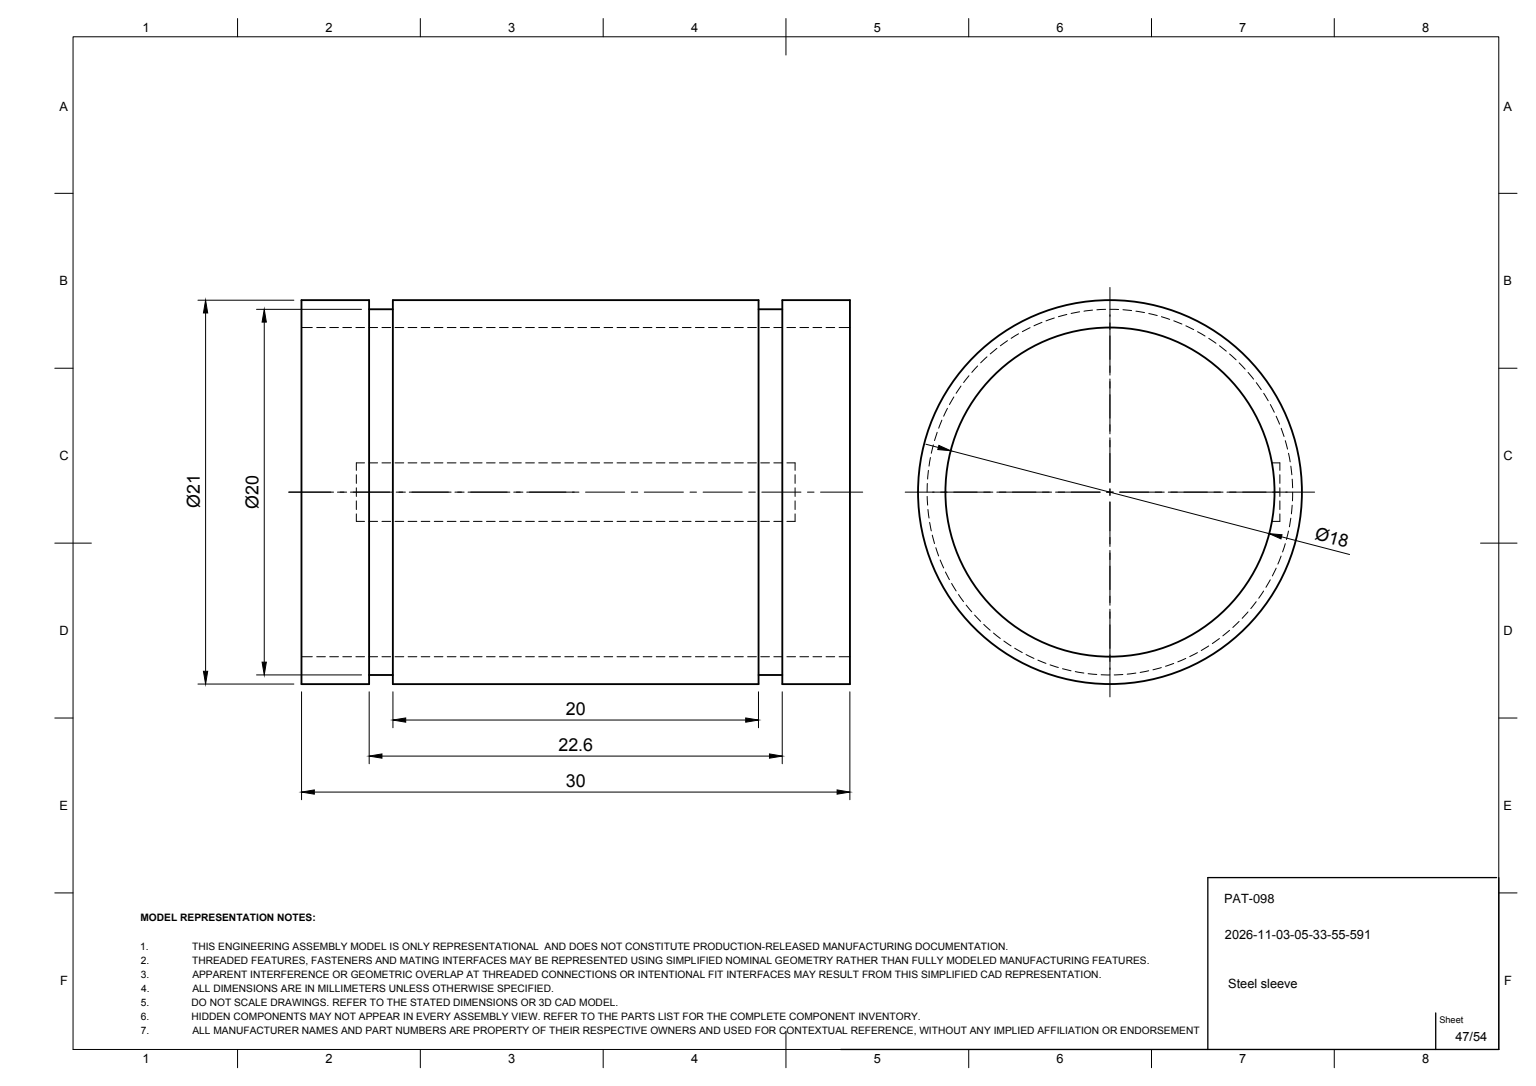
ISO-10303-21;
HEADER;
/* Generated by software containing ST-Developer
 * from STEP Tools, Inc. (www.steptools.com) 
 */

FILE_DESCRIPTION(
/* description */ ('Spring compression tester'),
/* implementation_level */ '2;1');

FILE_NAME(
/* name */ 'Steel sleeve.step',
/* time_stamp */ '2026-10-28T03:24:11-07:00',
/* author */ (''),
/* organization */ (''),
/* preprocessor_version */ 'ST-DEVELOPER v20.2',
/* originating_system */ 'Autodesk Translation Framework v15.17.0.0',
/* authorisation */ '');

FILE_SCHEMA (('AUTOMOTIVE_DESIGN { 1 0 10303 214 3 1 1 }'));
ENDSEC;

DATA;
#10=MECHANICAL_DESIGN_GEOMETRIC_PRESENTATION_REPRESENTATION('',(#1164),#43521);
#1029=SHAPE_REPRESENTATION_RELATIONSHIP('SRR','None',#43845,#1089);
#1089=ADVANCED_BREP_SHAPE_REPRESENTATION('',(#1235),#43505);
#1164=STYLED_ITEM('',(#44216),#1235);
#1235=MANIFOLD_SOLID_BREP('Body1',#18605);
#1542=FACE_BOUND('',#4256,.T.);
#1543=FACE_BOUND('',#4259,.T.);
#1544=FACE_BOUND('',#4262,.T.);
#1545=FACE_BOUND('',#4265,.T.);
#1546=FACE_BOUND('',#4268,.T.);
#1547=FACE_BOUND('',#4271,.T.);
#1548=FACE_BOUND('',#4273,.T.);
#2066=PLANE('',#20641);
#2067=PLANE('',#20643);
#2068=PLANE('',#20644);
#2069=PLANE('',#20646);
#2070=PLANE('',#20647);
#2071=PLANE('',#20648);
#2072=PLANE('',#20653);
#2073=PLANE('',#20657);
#2074=PLANE('',#20661);
#2075=PLANE('',#20665);
#2076=PLANE('',#20669);
#2908=FACE_OUTER_BOUND('',#4250,.T.);
#2909=FACE_OUTER_BOUND('',#4251,.T.);
#2910=FACE_OUTER_BOUND('',#4252,.T.);
#2911=FACE_OUTER_BOUND('',#4253,.T.);
#2912=FACE_OUTER_BOUND('',#4254,.T.);
#2913=FACE_OUTER_BOUND('',#4255,.T.);
#2914=FACE_OUTER_BOUND('',#4257,.T.);
#2915=FACE_OUTER_BOUND('',#4258,.T.);
#2916=FACE_OUTER_BOUND('',#4260,.T.);
#2917=FACE_OUTER_BOUND('',#4261,.T.);
#2918=FACE_OUTER_BOUND('',#4263,.T.);
#2919=FACE_OUTER_BOUND('',#4264,.T.);
#2920=FACE_OUTER_BOUND('',#4266,.T.);
#2921=FACE_OUTER_BOUND('',#4267,.T.);
#2922=FACE_OUTER_BOUND('',#4269,.T.);
#2923=FACE_OUTER_BOUND('',#4270,.T.);
#2924=FACE_OUTER_BOUND('',#4272,.T.);
#4250=EDGE_LOOP('',(#15579,#15580,#15581,#15582));
#4251=EDGE_LOOP('',(#15583,#15584,#15585,#15586));
#4252=EDGE_LOOP('',(#15587,#15588,#15589,#15590));
#4253=EDGE_LOOP('',(#15591,#15592,#15593,#15594));
#4254=EDGE_LOOP('',(#15595,#15596,#15597,#15598));
#4255=EDGE_LOOP('',(#15599));
#4256=EDGE_LOOP('',(#15600));
#4257=EDGE_LOOP('',(#15601,#15602,#15603,#15604));
#4258=EDGE_LOOP('',(#15605));
#4259=EDGE_LOOP('',(#15606));
#4260=EDGE_LOOP('',(#15607,#15608,#15609,#15610));
#4261=EDGE_LOOP('',(#15611));
#4262=EDGE_LOOP('',(#15612));
#4263=EDGE_LOOP('',(#15613,#15614,#15615,#15616));
#4264=EDGE_LOOP('',(#15617));
#4265=EDGE_LOOP('',(#15618));
#4266=EDGE_LOOP('',(#15619,#15620,#15621,#15622));
#4267=EDGE_LOOP('',(#15623));
#4268=EDGE_LOOP('',(#15624));
#4269=EDGE_LOOP('',(#15625,#15626,#15627,#15628));
#4270=EDGE_LOOP('',(#15629));
#4271=EDGE_LOOP('',(#15630));
#4272=EDGE_LOOP('',(#15631,#15632,#15633,#15634));
#4273=EDGE_LOOP('',(#15635,#15636,#15637,#15638));
#5698=LINE('',#30702,#7130);
#5699=LINE('',#30704,#7131);
#5700=LINE('',#30705,#7132);
#5701=LINE('',#30708,#7133);
#5702=LINE('',#30710,#7134);
#5703=LINE('',#30711,#7135);
#5704=LINE('',#30716,#7136);
#5705=LINE('',#30717,#7137);
#5706=LINE('',#30719,#7138);
#5707=LINE('',#30720,#7139);
#5708=LINE('',#30730,#7140);
#5709=LINE('',#30737,#7141);
#5710=LINE('',#30744,#7142);
#5711=LINE('',#30751,#7143);
#5712=LINE('',#30758,#7144);
#5713=LINE('',#30763,#7145);
#7130=VECTOR('',#25006,1.);
#7131=VECTOR('',#25007,1.);
#7132=VECTOR('',#25008,1.);
#7133=VECTOR('',#25011,1.);
#7134=VECTOR('',#25012,1.);
#7135=VECTOR('',#25013,1.);
#7136=VECTOR('',#25018,1.);
#7137=VECTOR('',#25019,1.);
#7138=VECTOR('',#25022,1.);
#7139=VECTOR('',#25023,1.);
#7140=VECTOR('',#25036,1.05);
#7141=VECTOR('',#25045,1.);
#7142=VECTOR('',#25054,1.05);
#7143=VECTOR('',#25063,1.);
#7144=VECTOR('',#25072,1.05);
#7145=VECTOR('',#25079,0.9);
#8025=CIRCLE('',#20642,0.9);
#8026=CIRCLE('',#20645,0.9);
#8027=CIRCLE('',#20649,1.05);
#8028=CIRCLE('',#20650,0.9);
#8029=CIRCLE('',#20652,1.05);
#8030=CIRCLE('',#20654,1.);
#8031=CIRCLE('',#20656,1.);
#8032=CIRCLE('',#20658,1.05);
#8033=CIRCLE('',#20660,1.05);
#8034=CIRCLE('',#20662,1.);
#8035=CIRCLE('',#20664,1.);
#8036=CIRCLE('',#20666,1.05);
#8037=CIRCLE('',#20668,1.05);
#8038=CIRCLE('',#20670,0.9);
#9268=VERTEX_POINT('',#30698);
#9269=VERTEX_POINT('',#30699);
#9270=VERTEX_POINT('',#30701);
#9271=VERTEX_POINT('',#30703);
#9272=VERTEX_POINT('',#30707);
#9273=VERTEX_POINT('',#30709);
#9274=VERTEX_POINT('',#30713);
#9275=VERTEX_POINT('',#30715);
#9276=VERTEX_POINT('',#30723);
#9277=VERTEX_POINT('',#30725);
#9278=VERTEX_POINT('',#30728);
#9279=VERTEX_POINT('',#30732);
#9280=VERTEX_POINT('',#30735);
#9281=VERTEX_POINT('',#30739);
#9282=VERTEX_POINT('',#30742);
#9283=VERTEX_POINT('',#30746);
#9284=VERTEX_POINT('',#30749);
#9285=VERTEX_POINT('',#30753);
#9286=VERTEX_POINT('',#30756);
#9287=VERTEX_POINT('',#30760);
#11454=EDGE_CURVE('',#9268,#9269,#8025,.T.);
#11455=EDGE_CURVE('',#9270,#9268,#5698,.T.);
#11456=EDGE_CURVE('',#9271,#9270,#5699,.T.);
#11457=EDGE_CURVE('',#9269,#9271,#5700,.T.);
#11458=EDGE_CURVE('',#9269,#9272,#5701,.T.);
#11459=EDGE_CURVE('',#9273,#9271,#5702,.T.);
#11460=EDGE_CURVE('',#9273,#9272,#5703,.T.);
#11461=EDGE_CURVE('',#9272,#9274,#8026,.T.);
#11462=EDGE_CURVE('',#9275,#9273,#5704,.T.);
#11463=EDGE_CURVE('',#9274,#9275,#5705,.T.);
#11464=EDGE_CURVE('',#9274,#9268,#5706,.T.);
#11465=EDGE_CURVE('',#9275,#9270,#5707,.T.);
#11466=EDGE_CURVE('',#9276,#9276,#8027,.T.);
#11467=EDGE_CURVE('',#9277,#9277,#8028,.T.);
#11468=EDGE_CURVE('',#9278,#9278,#8029,.T.);
#11469=EDGE_CURVE('',#9278,#9276,#5708,.T.);
#11470=EDGE_CURVE('',#9279,#9279,#8030,.T.);
#11471=EDGE_CURVE('',#9280,#9280,#8031,.T.);
#11472=EDGE_CURVE('',#9280,#9279,#5709,.T.);
#11473=EDGE_CURVE('',#9281,#9281,#8032,.T.);
#11474=EDGE_CURVE('',#9282,#9282,#8033,.T.);
#11475=EDGE_CURVE('',#9282,#9281,#5710,.T.);
#11476=EDGE_CURVE('',#9283,#9283,#8034,.T.);
#11477=EDGE_CURVE('',#9284,#9284,#8035,.T.);
#11478=EDGE_CURVE('',#9284,#9283,#5711,.T.);
#11479=EDGE_CURVE('',#9285,#9285,#8036,.T.);
#11480=EDGE_CURVE('',#9286,#9286,#8037,.T.);
#11481=EDGE_CURVE('',#9286,#9285,#5712,.T.);
#11482=EDGE_CURVE('',#9287,#9287,#8038,.T.);
#11483=EDGE_CURVE('',#9287,#9277,#5713,.T.);
#15579=ORIENTED_EDGE('',*,*,#11454,.F.);
#15580=ORIENTED_EDGE('',*,*,#11455,.F.);
#15581=ORIENTED_EDGE('',*,*,#11456,.F.);
#15582=ORIENTED_EDGE('',*,*,#11457,.F.);
#15583=ORIENTED_EDGE('',*,*,#11458,.F.);
#15584=ORIENTED_EDGE('',*,*,#11457,.T.);
#15585=ORIENTED_EDGE('',*,*,#11459,.F.);
#15586=ORIENTED_EDGE('',*,*,#11460,.T.);
#15587=ORIENTED_EDGE('',*,*,#11461,.F.);
#15588=ORIENTED_EDGE('',*,*,#11460,.F.);
#15589=ORIENTED_EDGE('',*,*,#11462,.F.);
#15590=ORIENTED_EDGE('',*,*,#11463,.F.);
#15591=ORIENTED_EDGE('',*,*,#11464,.F.);
#15592=ORIENTED_EDGE('',*,*,#11463,.T.);
#15593=ORIENTED_EDGE('',*,*,#11465,.T.);
#15594=ORIENTED_EDGE('',*,*,#11455,.T.);
#15595=ORIENTED_EDGE('',*,*,#11465,.F.);
#15596=ORIENTED_EDGE('',*,*,#11462,.T.);
#15597=ORIENTED_EDGE('',*,*,#11459,.T.);
#15598=ORIENTED_EDGE('',*,*,#11456,.T.);
#15599=ORIENTED_EDGE('',*,*,#11466,.F.);
#15600=ORIENTED_EDGE('',*,*,#11467,.T.);
#15601=ORIENTED_EDGE('',*,*,#11468,.F.);
#15602=ORIENTED_EDGE('',*,*,#11469,.T.);
#15603=ORIENTED_EDGE('',*,*,#11466,.T.);
#15604=ORIENTED_EDGE('',*,*,#11469,.F.);
#15605=ORIENTED_EDGE('',*,*,#11468,.T.);
#15606=ORIENTED_EDGE('',*,*,#11470,.F.);
#15607=ORIENTED_EDGE('',*,*,#11471,.F.);
#15608=ORIENTED_EDGE('',*,*,#11472,.T.);
#15609=ORIENTED_EDGE('',*,*,#11470,.T.);
#15610=ORIENTED_EDGE('',*,*,#11472,.F.);
#15611=ORIENTED_EDGE('',*,*,#11473,.F.);
#15612=ORIENTED_EDGE('',*,*,#11471,.T.);
#15613=ORIENTED_EDGE('',*,*,#11474,.F.);
#15614=ORIENTED_EDGE('',*,*,#11475,.T.);
#15615=ORIENTED_EDGE('',*,*,#11473,.T.);
#15616=ORIENTED_EDGE('',*,*,#11475,.F.);
#15617=ORIENTED_EDGE('',*,*,#11474,.T.);
#15618=ORIENTED_EDGE('',*,*,#11476,.F.);
#15619=ORIENTED_EDGE('',*,*,#11477,.F.);
#15620=ORIENTED_EDGE('',*,*,#11478,.T.);
#15621=ORIENTED_EDGE('',*,*,#11476,.T.);
#15622=ORIENTED_EDGE('',*,*,#11478,.F.);
#15623=ORIENTED_EDGE('',*,*,#11479,.F.);
#15624=ORIENTED_EDGE('',*,*,#11477,.T.);
#15625=ORIENTED_EDGE('',*,*,#11480,.F.);
#15626=ORIENTED_EDGE('',*,*,#11481,.T.);
#15627=ORIENTED_EDGE('',*,*,#11479,.T.);
#15628=ORIENTED_EDGE('',*,*,#11481,.F.);
#15629=ORIENTED_EDGE('',*,*,#11480,.T.);
#15630=ORIENTED_EDGE('',*,*,#11482,.F.);
#15631=ORIENTED_EDGE('',*,*,#11482,.T.);
#15632=ORIENTED_EDGE('',*,*,#11483,.T.);
#15633=ORIENTED_EDGE('',*,*,#11467,.F.);
#15634=ORIENTED_EDGE('',*,*,#11483,.F.);
#15635=ORIENTED_EDGE('',*,*,#11461,.T.);
#15636=ORIENTED_EDGE('',*,*,#11464,.T.);
#15637=ORIENTED_EDGE('',*,*,#11454,.T.);
#15638=ORIENTED_EDGE('',*,*,#11458,.T.);
#17306=CYLINDRICAL_SURFACE('',#20651,1.05);
#17307=CYLINDRICAL_SURFACE('',#20655,1.);
#17308=CYLINDRICAL_SURFACE('',#20659,1.05);
#17309=CYLINDRICAL_SURFACE('',#20663,1.);
#17310=CYLINDRICAL_SURFACE('',#20667,1.05);
#17311=CYLINDRICAL_SURFACE('',#20671,0.9);
#18232=ADVANCED_FACE('',(#2908),#2066,.F.);
#18233=ADVANCED_FACE('',(#2909),#2067,.F.);
#18234=ADVANCED_FACE('',(#2910),#2068,.F.);
#18235=ADVANCED_FACE('',(#2911),#2069,.F.);
#18236=ADVANCED_FACE('',(#2912),#2070,.F.);
#18237=ADVANCED_FACE('',(#2913,#1542),#2071,.T.);
#18238=ADVANCED_FACE('',(#2914),#17306,.T.);
#18239=ADVANCED_FACE('',(#2915,#1543),#2072,.T.);
#18240=ADVANCED_FACE('',(#2916),#17307,.T.);
#18241=ADVANCED_FACE('',(#2917,#1544),#2073,.T.);
#18242=ADVANCED_FACE('',(#2918),#17308,.T.);
#18243=ADVANCED_FACE('',(#2919,#1545),#2074,.T.);
#18244=ADVANCED_FACE('',(#2920),#17309,.T.);
#18245=ADVANCED_FACE('',(#2921,#1546),#2075,.T.);
#18246=ADVANCED_FACE('',(#2922),#17310,.T.);
#18247=ADVANCED_FACE('',(#2923,#1547),#2076,.T.);
#18248=ADVANCED_FACE('',(#2924,#1548),#17311,.F.);
#18605=CLOSED_SHELL('',(#18232,#18233,#18234,#18235,#18236,#18237,#18238,
#18239,#18240,#18241,#18242,#18243,#18244,#18245,#18246,#18247,#18248));
#20640=AXIS2_PLACEMENT_3D('',#30696,#25000,#25001);
#20641=AXIS2_PLACEMENT_3D('',#30697,#25002,#25003);
#20642=AXIS2_PLACEMENT_3D('',#30700,#25004,#25005);
#20643=AXIS2_PLACEMENT_3D('',#30706,#25009,#25010);
#20644=AXIS2_PLACEMENT_3D('',#30712,#25014,#25015);
#20645=AXIS2_PLACEMENT_3D('',#30714,#25016,#25017);
#20646=AXIS2_PLACEMENT_3D('',#30718,#25020,#25021);
#20647=AXIS2_PLACEMENT_3D('',#30721,#25024,#25025);
#20648=AXIS2_PLACEMENT_3D('',#30722,#25026,#25027);
#20649=AXIS2_PLACEMENT_3D('',#30724,#25028,#25029);
#20650=AXIS2_PLACEMENT_3D('',#30726,#25030,#25031);
#20651=AXIS2_PLACEMENT_3D('',#30727,#25032,#25033);
#20652=AXIS2_PLACEMENT_3D('',#30729,#25034,#25035);
#20653=AXIS2_PLACEMENT_3D('',#30731,#25037,#25038);
#20654=AXIS2_PLACEMENT_3D('',#30733,#25039,#25040);
#20655=AXIS2_PLACEMENT_3D('',#30734,#25041,#25042);
#20656=AXIS2_PLACEMENT_3D('',#30736,#25043,#25044);
#20657=AXIS2_PLACEMENT_3D('',#30738,#25046,#25047);
#20658=AXIS2_PLACEMENT_3D('',#30740,#25048,#25049);
#20659=AXIS2_PLACEMENT_3D('',#30741,#25050,#25051);
#20660=AXIS2_PLACEMENT_3D('',#30743,#25052,#25053);
#20661=AXIS2_PLACEMENT_3D('',#30745,#25055,#25056);
#20662=AXIS2_PLACEMENT_3D('',#30747,#25057,#25058);
#20663=AXIS2_PLACEMENT_3D('',#30748,#25059,#25060);
#20664=AXIS2_PLACEMENT_3D('',#30750,#25061,#25062);
#20665=AXIS2_PLACEMENT_3D('',#30752,#25064,#25065);
#20666=AXIS2_PLACEMENT_3D('',#30754,#25066,#25067);
#20667=AXIS2_PLACEMENT_3D('',#30755,#25068,#25069);
#20668=AXIS2_PLACEMENT_3D('',#30757,#25070,#25071);
#20669=AXIS2_PLACEMENT_3D('',#30759,#25073,#25074);
#20670=AXIS2_PLACEMENT_3D('',#30761,#25075,#25076);
#20671=AXIS2_PLACEMENT_3D('',#30762,#25077,#25078);
#25000=DIRECTION('axis',(0.,0.,1.));
#25001=DIRECTION('refdir',(1.,0.,0.));
#25002=DIRECTION('center_axis',(0.,1.,0.));
#25003=DIRECTION('ref_axis',(0.,0.,1.));
#25004=DIRECTION('center_axis',(0.,-1.,0.));
#25005=DIRECTION('ref_axis',(1.,0.,0.));
#25006=DIRECTION('',(-1.,0.,0.));
#25007=DIRECTION('',(0.,0.,-1.));
#25008=DIRECTION('',(1.,0.,0.));
#25009=DIRECTION('center_axis',(0.,0.,1.));
#25010=DIRECTION('ref_axis',(1.,0.,0.));
#25011=DIRECTION('',(0.,-1.,0.));
#25012=DIRECTION('',(0.,1.,0.));
#25013=DIRECTION('',(-1.,0.,0.));
#25014=DIRECTION('center_axis',(0.,-1.,0.));
#25015=DIRECTION('ref_axis',(0.,0.,-1.));
#25016=DIRECTION('center_axis',(0.,1.,0.));
#25017=DIRECTION('ref_axis',(1.,0.,0.));
#25018=DIRECTION('',(0.,0.,1.));
#25019=DIRECTION('',(1.,0.,0.));
#25020=DIRECTION('center_axis',(0.,0.,-1.));
#25021=DIRECTION('ref_axis',(-1.,0.,0.));
#25022=DIRECTION('',(0.,1.,0.));
#25023=DIRECTION('',(0.,1.,0.));
#25024=DIRECTION('center_axis',(1.,0.,0.));
#25025=DIRECTION('ref_axis',(0.,0.,-1.));
#25026=DIRECTION('center_axis',(0.,1.,0.));
#25027=DIRECTION('ref_axis',(0.,0.,1.));
#25028=DIRECTION('center_axis',(0.,-1.,0.));
#25029=DIRECTION('ref_axis',(1.,0.,0.));
#25030=DIRECTION('center_axis',(0.,-1.,0.));
#25031=DIRECTION('ref_axis',(1.,0.,0.));
#25032=DIRECTION('center_axis',(0.,-1.,0.));
#25033=DIRECTION('ref_axis',(1.,0.,0.));
#25034=DIRECTION('center_axis',(0.,-1.,0.));
#25035=DIRECTION('ref_axis',(1.,0.,0.));
#25036=DIRECTION('',(0.,1.,0.));
#25037=DIRECTION('center_axis',(0.,-1.,0.));
#25038=DIRECTION('ref_axis',(0.,0.,-1.));
#25039=DIRECTION('center_axis',(0.,-1.,0.));
#25040=DIRECTION('ref_axis',(1.,0.,0.));
#25041=DIRECTION('center_axis',(0.,-1.,0.));
#25042=DIRECTION('ref_axis',(1.,0.,0.));
#25043=DIRECTION('center_axis',(0.,-1.,0.));
#25044=DIRECTION('ref_axis',(1.,0.,0.));
#25045=DIRECTION('',(0.,1.,0.));
#25046=DIRECTION('center_axis',(0.,1.,0.));
#25047=DIRECTION('ref_axis',(0.,0.,1.));
#25048=DIRECTION('center_axis',(0.,-1.,0.));
#25049=DIRECTION('ref_axis',(1.,0.,0.));
#25050=DIRECTION('center_axis',(0.,-1.,0.));
#25051=DIRECTION('ref_axis',(1.,0.,0.));
#25052=DIRECTION('center_axis',(0.,-1.,0.));
#25053=DIRECTION('ref_axis',(1.,0.,0.));
#25054=DIRECTION('',(0.,1.,0.));
#25055=DIRECTION('center_axis',(0.,-1.,0.));
#25056=DIRECTION('ref_axis',(0.,0.,-1.));
#25057=DIRECTION('center_axis',(0.,-1.,0.));
#25058=DIRECTION('ref_axis',(1.,0.,0.));
#25059=DIRECTION('center_axis',(0.,-1.,0.));
#25060=DIRECTION('ref_axis',(1.,0.,0.));
#25061=DIRECTION('center_axis',(0.,-1.,0.));
#25062=DIRECTION('ref_axis',(1.,0.,0.));
#25063=DIRECTION('',(0.,1.,0.));
#25064=DIRECTION('center_axis',(0.,1.,0.));
#25065=DIRECTION('ref_axis',(0.,0.,1.));
#25066=DIRECTION('center_axis',(0.,-1.,0.));
#25067=DIRECTION('ref_axis',(1.,0.,0.));
#25068=DIRECTION('center_axis',(0.,-1.,0.));
#25069=DIRECTION('ref_axis',(1.,0.,0.));
#25070=DIRECTION('center_axis',(0.,-1.,0.));
#25071=DIRECTION('ref_axis',(1.,0.,0.));
#25072=DIRECTION('',(0.,1.,0.));
#25073=DIRECTION('center_axis',(0.,-1.,0.));
#25074=DIRECTION('ref_axis',(0.,0.,-1.));
#25075=DIRECTION('center_axis',(0.,-1.,0.));
#25076=DIRECTION('ref_axis',(1.,0.,0.));
#25077=DIRECTION('center_axis',(0.,-1.,0.));
#25078=DIRECTION('ref_axis',(1.,0.,0.));
#25079=DIRECTION('',(0.,1.,0.));
#30696=CARTESIAN_POINT('',(0.,0.,0.));
#30697=CARTESIAN_POINT('Origin',(0.75,1.2,0.));
#30698=CARTESIAN_POINT('',(0.885663593019381,1.2,-0.16));
#30699=CARTESIAN_POINT('',(0.885663593019381,1.2,0.16));
#30700=CARTESIAN_POINT('Origin',(0.,1.2,0.));
#30701=CARTESIAN_POINT('',(0.93,1.2,-0.16));
#30702=CARTESIAN_POINT('',(0.93,1.2,-0.16));
#30703=CARTESIAN_POINT('',(0.93,1.2,0.16));
#30704=CARTESIAN_POINT('',(0.93,1.2,0.16));
#30705=CARTESIAN_POINT('',(0.57,1.2,0.16));
#30706=CARTESIAN_POINT('Origin',(0.57,0.,0.16));
#30707=CARTESIAN_POINT('',(0.885663593019381,-1.2,0.16));
#30708=CARTESIAN_POINT('',(0.885663593019381,0.,0.16));
#30709=CARTESIAN_POINT('',(0.93,-1.2,0.16));
#30710=CARTESIAN_POINT('',(0.93,0.,0.16));
#30711=CARTESIAN_POINT('',(0.57,-1.2,0.16));
#30712=CARTESIAN_POINT('Origin',(0.75,-1.2,0.));
#30713=CARTESIAN_POINT('',(0.885663593019381,-1.2,-0.16));
#30714=CARTESIAN_POINT('Origin',(0.,-1.2,0.));
#30715=CARTESIAN_POINT('',(0.93,-1.2,-0.16));
#30716=CARTESIAN_POINT('',(0.93,-1.2,0.16));
#30717=CARTESIAN_POINT('',(0.93,-1.2,-0.16));
#30718=CARTESIAN_POINT('Origin',(0.93,0.,-0.16));
#30719=CARTESIAN_POINT('',(0.885663593019381,0.,-0.16));
#30720=CARTESIAN_POINT('',(0.93,0.,-0.16));
#30721=CARTESIAN_POINT('Origin',(0.93,0.,0.16));
#30722=CARTESIAN_POINT('Origin',(1.05,1.5,0.));
#30723=CARTESIAN_POINT('',(-1.05,1.5,-1.28587913910472E-16));
#30724=CARTESIAN_POINT('Origin',(0.,1.5,0.));
#30725=CARTESIAN_POINT('',(-0.9,1.5,-1.10218211923262E-16));
#30726=CARTESIAN_POINT('Origin',(0.,1.5,0.));
#30727=CARTESIAN_POINT('Origin',(0.,1.315,0.));
#30728=CARTESIAN_POINT('',(-1.05,1.13,-1.28587913910472E-16));
#30729=CARTESIAN_POINT('Origin',(0.,1.13,0.));
#30730=CARTESIAN_POINT('',(-1.05,1.315,-1.28587913910472E-16));
#30731=CARTESIAN_POINT('Origin',(1.,1.13,0.));
#30732=CARTESIAN_POINT('',(-1.,1.13,-1.22464679914735E-16));
#30733=CARTESIAN_POINT('Origin',(0.,1.13,0.));
#30734=CARTESIAN_POINT('Origin',(0.,1.065,0.));
#30735=CARTESIAN_POINT('',(-1.,1.,-1.22464679914735E-16));
#30736=CARTESIAN_POINT('Origin',(0.,1.,0.));
#30737=CARTESIAN_POINT('',(-1.,1.065,-1.22464679914735E-16));
#30738=CARTESIAN_POINT('Origin',(1.05,1.,0.));
#30739=CARTESIAN_POINT('',(-1.05,1.,-1.28587913910472E-16));
#30740=CARTESIAN_POINT('Origin',(0.,1.,0.));
#30741=CARTESIAN_POINT('Origin',(0.,0.,0.));
#30742=CARTESIAN_POINT('',(-1.05,-1.,-1.28587913910472E-16));
#30743=CARTESIAN_POINT('Origin',(0.,-1.,0.));
#30744=CARTESIAN_POINT('',(-1.05,0.,-1.28587913910472E-16));
#30745=CARTESIAN_POINT('Origin',(1.,-1.,0.));
#30746=CARTESIAN_POINT('',(-1.,-1.,-1.22464679914735E-16));
#30747=CARTESIAN_POINT('Origin',(0.,-1.,0.));
#30748=CARTESIAN_POINT('Origin',(0.,-1.065,0.));
#30749=CARTESIAN_POINT('',(-1.,-1.13,-1.22464679914735E-16));
#30750=CARTESIAN_POINT('Origin',(0.,-1.13,0.));
#30751=CARTESIAN_POINT('',(-1.,-1.065,-1.22464679914735E-16));
#30752=CARTESIAN_POINT('Origin',(1.05,-1.13,0.));
#30753=CARTESIAN_POINT('',(-1.05,-1.13,-1.28587913910472E-16));
#30754=CARTESIAN_POINT('Origin',(0.,-1.13,0.));
#30755=CARTESIAN_POINT('Origin',(0.,-1.315,0.));
#30756=CARTESIAN_POINT('',(-1.05,-1.5,-1.28587913910472E-16));
#30757=CARTESIAN_POINT('Origin',(0.,-1.5,0.));
#30758=CARTESIAN_POINT('',(-1.05,-1.315,-1.28587913910472E-16));
#30759=CARTESIAN_POINT('Origin',(0.9,-1.5,0.));
#30760=CARTESIAN_POINT('',(-0.9,-1.5,-1.10218211923262E-16));
#30761=CARTESIAN_POINT('Origin',(0.,-1.5,0.));
#30762=CARTESIAN_POINT('Origin',(0.,0.,0.));
#30763=CARTESIAN_POINT('',(-0.9,0.,-1.10218211923262E-16));
#43437=UNCERTAINTY_MEASURE_WITH_UNIT(LENGTH_MEASURE(0.001),#43522,
'DISTANCE_ACCURACY_VALUE',
'Maximum model space distance between geometric entities at asserted c
onnectivities');
#43453=UNCERTAINTY_MEASURE_WITH_UNIT(LENGTH_MEASURE(0.001),#43522,
'DISTANCE_ACCURACY_VALUE',
'Maximum model space distance between geometric entities at asserted c
onnectivities');
#43505=(
GEOMETRIC_REPRESENTATION_CONTEXT(3)
GLOBAL_UNCERTAINTY_ASSIGNED_CONTEXT((#43437))
GLOBAL_UNIT_ASSIGNED_CONTEXT((#43522,#43524,#43525))
REPRESENTATION_CONTEXT('','3D')
);
#43521=(
GEOMETRIC_REPRESENTATION_CONTEXT(3)
GLOBAL_UNCERTAINTY_ASSIGNED_CONTEXT((#43453))
GLOBAL_UNIT_ASSIGNED_CONTEXT((#43522,#43524,#43525))
REPRESENTATION_CONTEXT('','3D')
);
#43522=(
LENGTH_UNIT()
NAMED_UNIT(*)
SI_UNIT(.CENTI.,.METRE.)
);
#43524=(
NAMED_UNIT(*)
PLANE_ANGLE_UNIT()
SI_UNIT($,.RADIAN.)
);
#43525=(
NAMED_UNIT(*)
SI_UNIT($,.STERADIAN.)
SOLID_ANGLE_UNIT()
);
#43577=SHAPE_DEFINITION_REPRESENTATION(#43654,#43845);
#43654=PRODUCT_DEFINITION_SHAPE('',$,#43913);
#43845=SHAPE_REPRESENTATION('',(#20640),#43505);
#43861=PRODUCT_DEFINITION_CONTEXT('part definition',#44064,'design');
#43913=PRODUCT_DEFINITION('Steel sleeve','Steel sleeve',#43980,#43861);
#43980=PRODUCT_DEFINITION_FORMATION('',$,#44117);
#44064=APPLICATION_CONTEXT(
'Core Data for Automotive Mechanical Design Process');
#44065=PRODUCT_CONTEXT('part definition',#44064,'mechanical');
#44117=PRODUCT('Steel sleeve','Steel sleeve','Steel sleeve',(#44065));
#44210=COLOUR_RGB('Off White',0.89,0.88,0.83);
#44211=FILL_AREA_STYLE_COLOUR('',#44210);
#44212=FILL_AREA_STYLE('',(#44211));
#44213=SURFACE_STYLE_FILL_AREA(#44212);
#44214=SURFACE_SIDE_STYLE('',(#44213));
#44215=SURFACE_STYLE_USAGE(.BOTH.,#44214);
#44216=PRESENTATION_STYLE_ASSIGNMENT((#44215));
ENDSEC;
END-ISO-10303-21;
